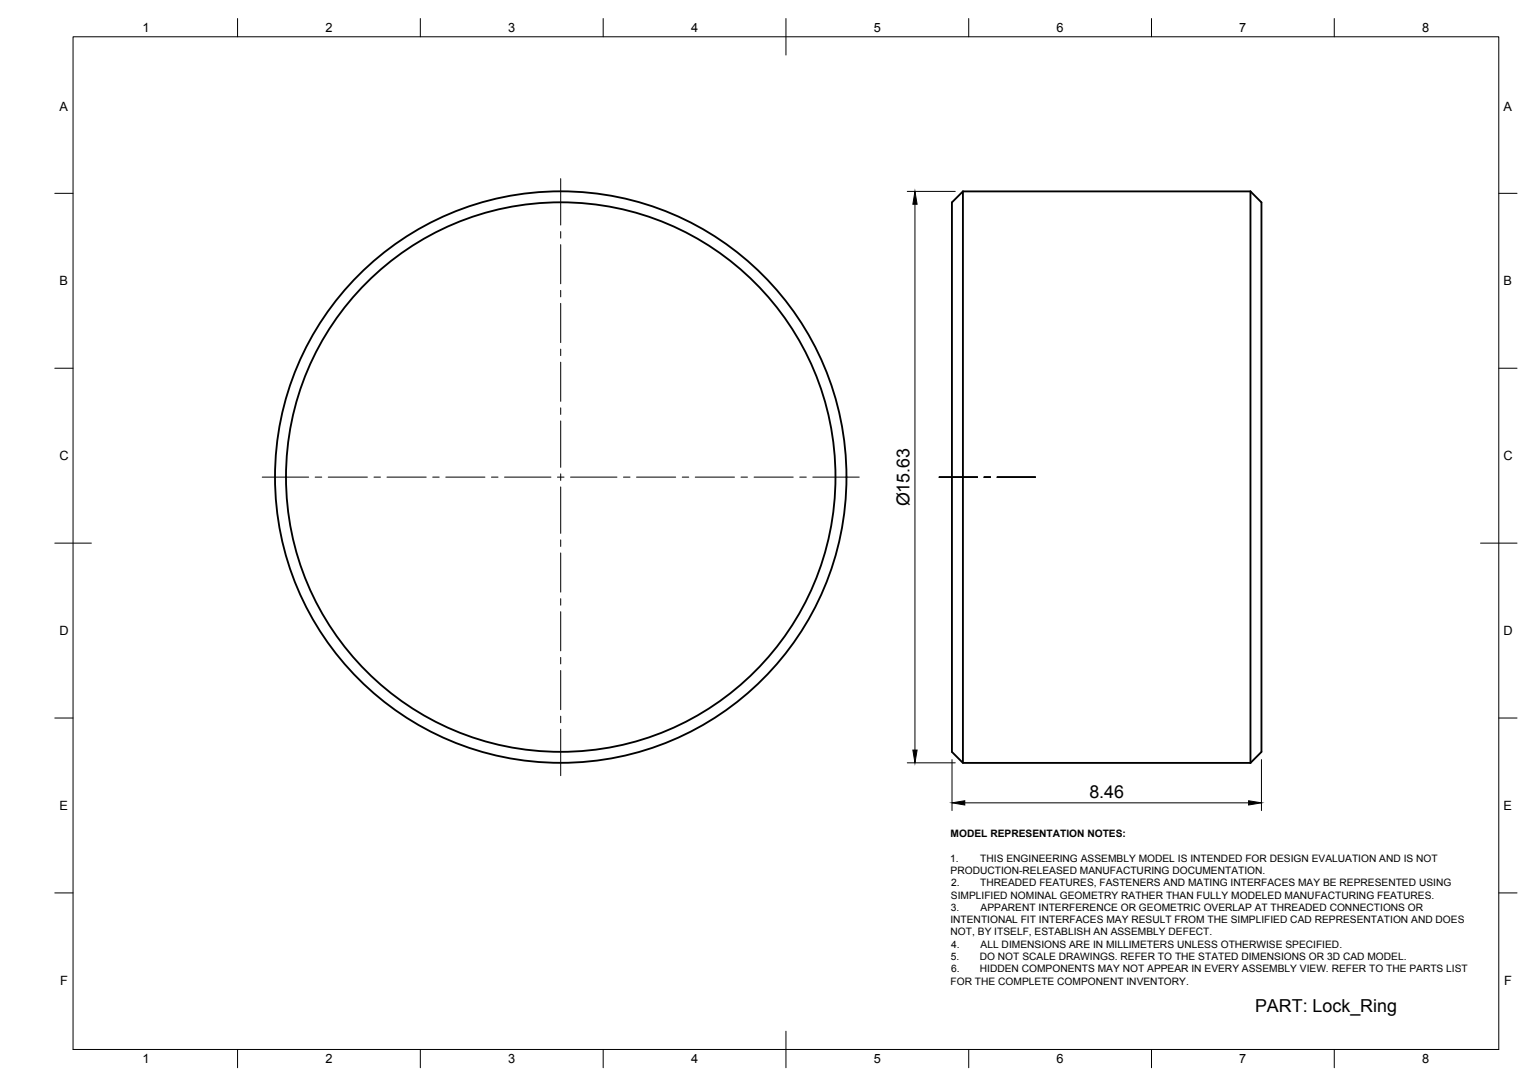
ISO-10303-21;
HEADER;
/* Generated by software containing ST-Developer
 * from STEP Tools, Inc. (www.steptools.com) 
 */

FILE_DESCRIPTION(
/* description */ (''),
/* implementation_level */ '2;1');

FILE_NAME(
/* name */ 'Lock_Ring.step',
/* time_stamp */ '2026-10-05T01:33:24-07:00',
/* author */ (''),
/* organization */ (''),
/* preprocessor_version */ 'ST-DEVELOPER v20.2',
/* originating_system */ 'Autodesk Translation Framework v15.15.0.0',
/* authorisation */ '');

FILE_SCHEMA (('AUTOMOTIVE_DESIGN { 1 0 10303 214 3 1 1 }'));
ENDSEC;

DATA;
#10=MECHANICAL_DESIGN_GEOMETRIC_PRESENTATION_REPRESENTATION('',(#90),#1128);
#60=CONICAL_SURFACE('',#714,7.66499874644978,0.785398163397445);
#61=CONICAL_SURFACE('',#722,7.66499874644978,0.785398163397452);
#70=SHAPE_REPRESENTATION_RELATIONSHIP('SRR','None',#1174,#80);
#80=ADVANCED_BREP_SHAPE_REPRESENTATION('',(#100),#1126);
#90=STYLED_ITEM('',(#1225),#100);
#100=MANIFOLD_SOLID_BREP('Body1',#529);
#115=LINE('',#1071,#132);
#116=LINE('',#1076,#133);
#117=LINE('',#1083,#134);
#132=VECTOR('',#902,7.66499874644978);
#133=VECTOR('',#909,7.81499874644978);
#134=VECTOR('',#918,7.66499874644978);
#144=CYLINDRICAL_SURFACE('',#718,7.81499874644978);
#179=FACE_OUTER_BOUND('',#220,.T.);
#180=FACE_OUTER_BOUND('',#221,.T.);
#181=FACE_OUTER_BOUND('',#222,.T.);
#182=FACE_OUTER_BOUND('',#223,.T.);
#183=FACE_OUTER_BOUND('',#224,.T.);
#220=EDGE_LOOP('',(#436,#437,#438,#439,#440));
#221=EDGE_LOOP('',(#441,#442,#443,#444,#445,#446));
#222=EDGE_LOOP('',(#447));
#223=EDGE_LOOP('',(#448,#449,#450,#451,#452));
#224=EDGE_LOOP('',(#453));
#257=CIRCLE('',#715,7.81499874644978);
#258=CIRCLE('',#716,7.51499874644978);
#259=CIRCLE('',#717,7.81499874644978);
#260=CIRCLE('',#719,7.81499874644978);
#261=CIRCLE('',#720,7.81499874644978);
#262=CIRCLE('',#723,7.51499874644978);
#290=VERTEX_POINT('',#1067);
#291=VERTEX_POINT('',#1068);
#292=VERTEX_POINT('',#1070);
#293=VERTEX_POINT('',#1075);
#294=VERTEX_POINT('',#1077);
#295=VERTEX_POINT('',#1082);
#340=EDGE_CURVE('',#290,#291,#257,.T.);
#341=EDGE_CURVE('',#291,#292,#115,.T.);
#342=EDGE_CURVE('',#292,#292,#258,.T.);
#343=EDGE_CURVE('',#291,#290,#259,.T.);
#344=EDGE_CURVE('',#290,#293,#116,.T.);
#345=EDGE_CURVE('',#294,#293,#260,.T.);
#346=EDGE_CURVE('',#293,#294,#261,.T.);
#347=EDGE_CURVE('',#294,#295,#117,.T.);
#348=EDGE_CURVE('',#295,#295,#262,.T.);
#436=ORIENTED_EDGE('',*,*,#340,.T.);
#437=ORIENTED_EDGE('',*,*,#341,.T.);
#438=ORIENTED_EDGE('',*,*,#342,.T.);
#439=ORIENTED_EDGE('',*,*,#341,.F.);
#440=ORIENTED_EDGE('',*,*,#343,.T.);
#441=ORIENTED_EDGE('',*,*,#340,.F.);
#442=ORIENTED_EDGE('',*,*,#344,.T.);
#443=ORIENTED_EDGE('',*,*,#345,.F.);
#444=ORIENTED_EDGE('',*,*,#346,.F.);
#445=ORIENTED_EDGE('',*,*,#344,.F.);
#446=ORIENTED_EDGE('',*,*,#343,.F.);
#447=ORIENTED_EDGE('',*,*,#342,.F.);
#448=ORIENTED_EDGE('',*,*,#345,.T.);
#449=ORIENTED_EDGE('',*,*,#346,.T.);
#450=ORIENTED_EDGE('',*,*,#347,.T.);
#451=ORIENTED_EDGE('',*,*,#348,.T.);
#452=ORIENTED_EDGE('',*,*,#347,.F.);
#453=ORIENTED_EDGE('',*,*,#348,.F.);
#476=PLANE('',#721);
#477=PLANE('',#724);
#513=ADVANCED_FACE('',(#179),#60,.T.);
#514=ADVANCED_FACE('',(#180),#144,.T.);
#515=ADVANCED_FACE('',(#181),#476,.T.);
#516=ADVANCED_FACE('',(#182),#61,.T.);
#517=ADVANCED_FACE('',(#183),#477,.T.);
#529=CLOSED_SHELL('',(#513,#514,#515,#516,#517));
#713=AXIS2_PLACEMENT_3D('',#1065,#896,#897);
#714=AXIS2_PLACEMENT_3D('',#1066,#898,#899);
#715=AXIS2_PLACEMENT_3D('',#1069,#900,#901);
#716=AXIS2_PLACEMENT_3D('',#1072,#903,#904);
#717=AXIS2_PLACEMENT_3D('',#1073,#905,#906);
#718=AXIS2_PLACEMENT_3D('',#1074,#907,#908);
#719=AXIS2_PLACEMENT_3D('',#1078,#910,#911);
#720=AXIS2_PLACEMENT_3D('',#1079,#912,#913);
#721=AXIS2_PLACEMENT_3D('',#1080,#914,#915);
#722=AXIS2_PLACEMENT_3D('',#1081,#916,#917);
#723=AXIS2_PLACEMENT_3D('',#1084,#919,#920);
#724=AXIS2_PLACEMENT_3D('',#1085,#921,#922);
#896=DIRECTION('axis',(0.,0.,1.));
#897=DIRECTION('refdir',(1.,0.,0.));
#898=DIRECTION('center_axis',(-1.,0.,0.));
#899=DIRECTION('ref_axis',(0.,0.,1.));
#900=DIRECTION('center_axis',(1.,0.,0.));
#901=DIRECTION('ref_axis',(0.,0.,1.));
#902=DIRECTION('',(0.70710678118655,8.6595605623549E-17,0.707106781186545));
#903=DIRECTION('center_axis',(-1.,0.,0.));
#904=DIRECTION('ref_axis',(0.,0.,1.));
#905=DIRECTION('center_axis',(1.,0.,0.));
#906=DIRECTION('ref_axis',(0.,0.,1.));
#907=DIRECTION('center_axis',(1.,0.,0.));
#908=DIRECTION('ref_axis',(0.,0.,-1.));
#909=DIRECTION('',(-1.,0.,0.));
#910=DIRECTION('center_axis',(-1.,0.,0.));
#911=DIRECTION('ref_axis',(0.,0.,1.));
#912=DIRECTION('center_axis',(-1.,0.,0.));
#913=DIRECTION('ref_axis',(0.,0.,1.));
#914=DIRECTION('center_axis',(1.,0.,0.));
#915=DIRECTION('ref_axis',(0.,0.,-1.));
#916=DIRECTION('center_axis',(1.,0.,0.));
#917=DIRECTION('ref_axis',(0.,0.,1.));
#918=DIRECTION('',(-0.707106781186545,-8.65956056235497E-17,0.70710678118655));
#919=DIRECTION('center_axis',(1.,0.,0.));
#920=DIRECTION('ref_axis',(0.,0.,1.));
#921=DIRECTION('center_axis',(-1.,0.,0.));
#922=DIRECTION('ref_axis',(0.,0.,1.));
#1065=CARTESIAN_POINT('',(0.,0.,0.));
#1066=CARTESIAN_POINT('Origin',(40.2408939752243,0.,0.));
#1067=CARTESIAN_POINT('',(40.0908939752243,-9.5706132001803E-16,7.81499874644978));
#1068=CARTESIAN_POINT('',(40.0908939752243,-9.5706132001803E-16,-7.81499874644978));
#1069=CARTESIAN_POINT('Origin',(40.0908939752243,0.,0.));
#1070=CARTESIAN_POINT('',(40.3908939752244,-9.2032191604361E-16,-7.51499874644978));
#1071=CARTESIAN_POINT('',(40.2408939752243,-9.3869161803082E-16,-7.66499874644978));
#1072=CARTESIAN_POINT('Origin',(40.3908939752244,0.,0.));
#1073=CARTESIAN_POINT('Origin',(40.0908939752243,0.,0.));
#1074=CARTESIAN_POINT('Origin',(36.1586650048583,0.,0.));
#1075=CARTESIAN_POINT('',(32.2264360344922,-9.5706132001803E-16,7.81499874644978));
#1076=CARTESIAN_POINT('',(36.1586650048583,-9.5706132001803E-16,7.81499874644978));
#1077=CARTESIAN_POINT('',(32.2264360344922,-9.5706132001803E-16,-7.81499874644978));
#1078=CARTESIAN_POINT('Origin',(32.2264360344922,0.,0.));
#1079=CARTESIAN_POINT('Origin',(32.2264360344922,0.,0.));
#1080=CARTESIAN_POINT('Origin',(40.3908939752244,0.,0.));
#1081=CARTESIAN_POINT('Origin',(32.0764360344922,0.,0.));
#1082=CARTESIAN_POINT('',(31.9264360344922,9.2032191604361E-16,-7.51499874644978));
#1083=CARTESIAN_POINT('',(32.0764360344922,9.3869161803082E-16,-7.66499874644978));
#1084=CARTESIAN_POINT('Origin',(31.9264360344922,0.,0.));
#1085=CARTESIAN_POINT('Origin',(31.9264360344922,0.,-7.81499874644978));
#1114=UNCERTAINTY_MEASURE_WITH_UNIT(LENGTH_MEASURE(0.01),#1129,
'DISTANCE_ACCURACY_VALUE',
'Maximum model space distance between geometric entities at asserted c
onnectivities');
#1116=UNCERTAINTY_MEASURE_WITH_UNIT(LENGTH_MEASURE(0.01),#1129,
'DISTANCE_ACCURACY_VALUE',
'Maximum model space distance between geometric entities at asserted c
onnectivities');
#1126=(
GEOMETRIC_REPRESENTATION_CONTEXT(3)
GLOBAL_UNCERTAINTY_ASSIGNED_CONTEXT((#1114))
GLOBAL_UNIT_ASSIGNED_CONTEXT((#1129,#1131,#1132))
REPRESENTATION_CONTEXT('','3D')
);
#1128=(
GEOMETRIC_REPRESENTATION_CONTEXT(3)
GLOBAL_UNCERTAINTY_ASSIGNED_CONTEXT((#1116))
GLOBAL_UNIT_ASSIGNED_CONTEXT((#1129,#1131,#1132))
REPRESENTATION_CONTEXT('','3D')
);
#1129=(
LENGTH_UNIT()
NAMED_UNIT(*)
SI_UNIT(.MILLI.,.METRE.)
);
#1131=(
NAMED_UNIT(*)
PLANE_ANGLE_UNIT()
SI_UNIT($,.RADIAN.)
);
#1132=(
NAMED_UNIT(*)
SI_UNIT($,.STERADIAN.)
SOLID_ANGLE_UNIT()
);
#1142=SHAPE_DEFINITION_REPRESENTATION(#1153,#1174);
#1153=PRODUCT_DEFINITION_SHAPE('',$,#1186);
#1174=SHAPE_REPRESENTATION('',(#713),#1126);
#1176=PRODUCT_DEFINITION_CONTEXT('part definition',#1211,'design');
#1186=PRODUCT_DEFINITION('Lock_Ring','Lock_Ring',#1197,#1176);
#1197=PRODUCT_DEFINITION_FORMATION('',$,#1222);
#1211=APPLICATION_CONTEXT(
'Core Data for Automotive Mechanical Design Process');
#1212=PRODUCT_CONTEXT('part definition',#1211,'mechanical');
#1222=PRODUCT('Lock_Ring','Lock_Ring',$,(#1212));
#1225=PRESENTATION_STYLE_ASSIGNMENT((#1229));
#1229=SURFACE_STYLE_USAGE(.BOTH.,#1233);
#1233=SURFACE_SIDE_STYLE('',(#1237));
#1237=SURFACE_STYLE_FILL_AREA(#1241);
#1241=FILL_AREA_STYLE('Opaque(201,201,201)',(#1245));
#1245=FILL_AREA_STYLE_COLOUR('Opaque(201,201,201)',#1249);
#1249=COLOUR_RGB('Opaque(201,201,201)', 0.09019608, 0.27058824, 0.51372549);
ENDSEC;
END-ISO-10303-21;
